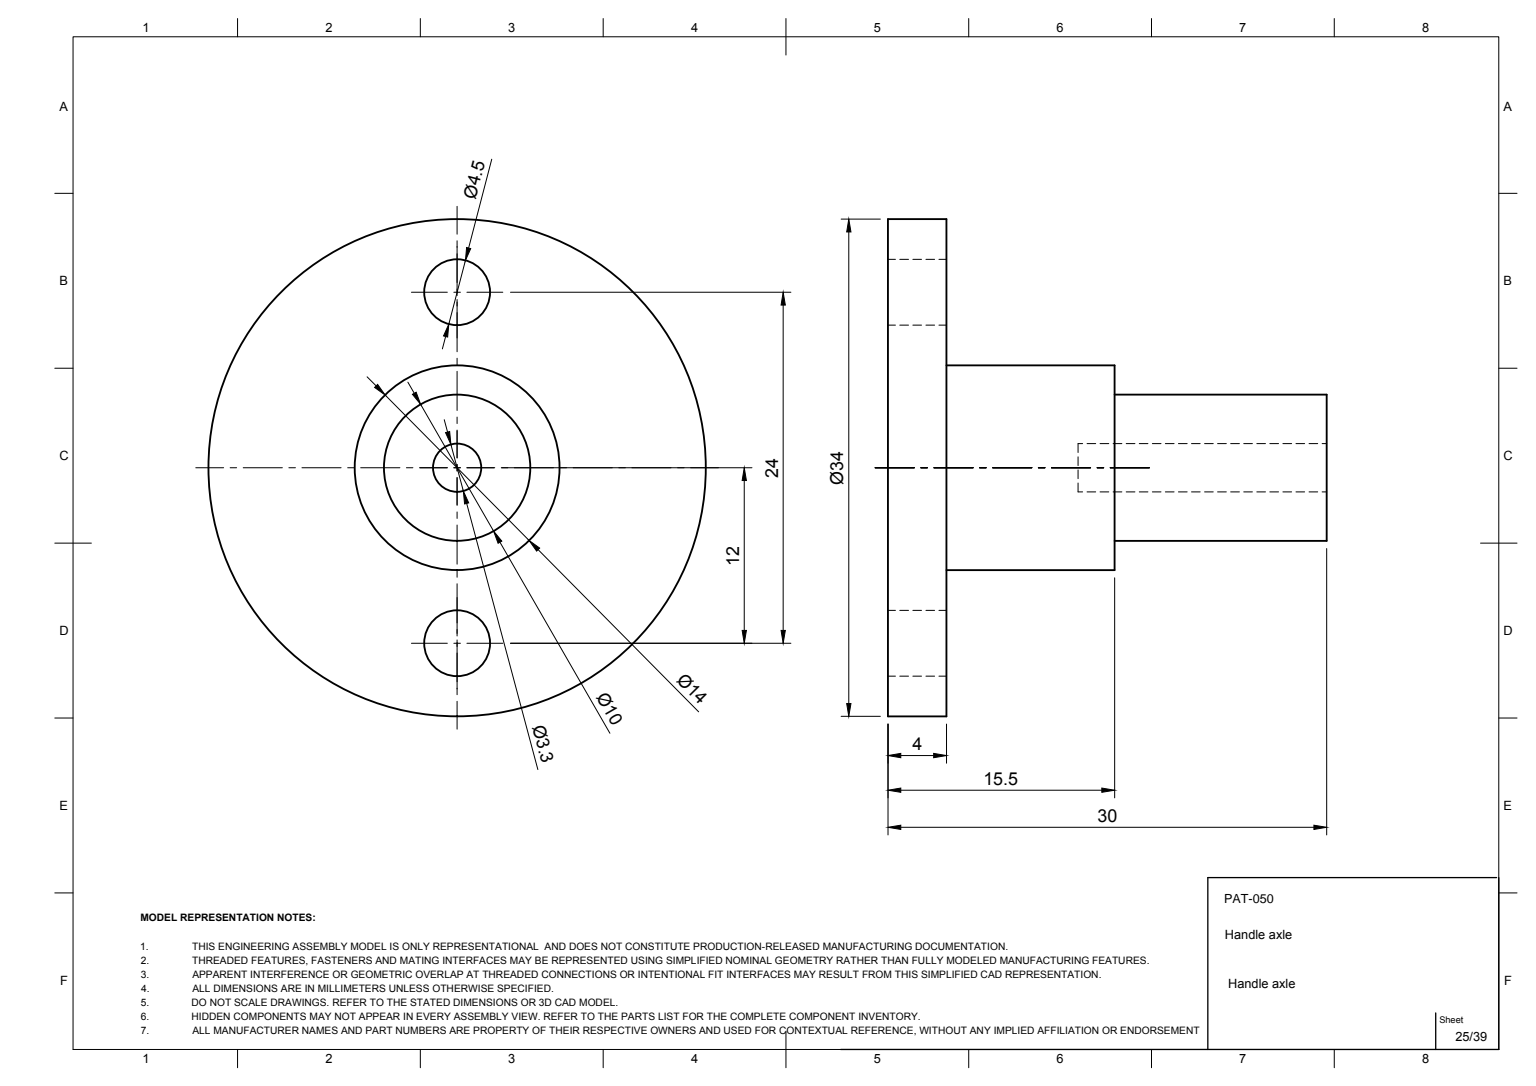
ISO-10303-21;
HEADER;
/* Generated by software containing ST-Developer
 * from STEP Tools, Inc. (www.steptools.com) 
 */

FILE_DESCRIPTION(
/* description */ ('Hand wheel with handle and shaft collar'),
/* implementation_level */ '2;1');

FILE_NAME(
/* name */ 'Handle axle.step',
/* time_stamp */ '2026-10-28T03:23:19-07:00',
/* author */ (''),
/* organization */ (''),
/* preprocessor_version */ 'ST-DEVELOPER v20.2',
/* originating_system */ 'Autodesk Translation Framework v15.17.0.0',
/* authorisation */ '');

FILE_SCHEMA (('AUTOMOTIVE_DESIGN { 1 0 10303 214 3 1 1 }'));
ENDSEC;

DATA;
#10=MECHANICAL_DESIGN_GEOMETRIC_PRESENTATION_REPRESENTATION('',(#420),#10510);
#349=SHAPE_REPRESENTATION_RELATIONSHIP('SRR','None',#10667,#381);
#381=ADVANCED_BREP_SHAPE_REPRESENTATION('',(#466),#10494);
#420=STYLED_ITEM('',(#10908),#466);
#466=MANIFOLD_SOLID_BREP('Body1',#5320);
#570=FACE_BOUND('',#1351,.T.);
#571=FACE_BOUND('',#1352,.T.);
#572=FACE_BOUND('',#1353,.T.);
#573=FACE_BOUND('',#1356,.T.);
#574=FACE_BOUND('',#1360,.T.);
#575=FACE_BOUND('',#1361,.T.);
#576=FACE_BOUND('',#1363,.T.);
#693=PLANE('',#6090);
#694=PLANE('',#6097);
#695=PLANE('',#6102);
#696=PLANE('',#6108);
#697=PLANE('',#6109);
#943=FACE_OUTER_BOUND('',#1346,.T.);
#944=FACE_OUTER_BOUND('',#1347,.T.);
#945=FACE_OUTER_BOUND('',#1348,.T.);
#946=FACE_OUTER_BOUND('',#1349,.T.);
#947=FACE_OUTER_BOUND('',#1350,.T.);
#948=FACE_OUTER_BOUND('',#1354,.T.);
#949=FACE_OUTER_BOUND('',#1355,.T.);
#950=FACE_OUTER_BOUND('',#1357,.T.);
#951=FACE_OUTER_BOUND('',#1358,.T.);
#952=FACE_OUTER_BOUND('',#1359,.T.);
#953=FACE_OUTER_BOUND('',#1362,.T.);
#1346=EDGE_LOOP('',(#4347,#4348,#4349,#4350));
#1347=EDGE_LOOP('',(#4351));
#1348=EDGE_LOOP('',(#4352,#4353,#4354,#4355));
#1349=EDGE_LOOP('',(#4356,#4357,#4358,#4359));
#1350=EDGE_LOOP('',(#4360));
#1351=EDGE_LOOP('',(#4361));
#1352=EDGE_LOOP('',(#4362));
#1353=EDGE_LOOP('',(#4363));
#1354=EDGE_LOOP('',(#4364,#4365,#4366,#4367));
#1355=EDGE_LOOP('',(#4368));
#1356=EDGE_LOOP('',(#4369));
#1357=EDGE_LOOP('',(#4370,#4371,#4372,#4373));
#1358=EDGE_LOOP('',(#4374,#4375,#4376,#4377));
#1359=EDGE_LOOP('',(#4378));
#1360=EDGE_LOOP('',(#4379));
#1361=EDGE_LOOP('',(#4380));
#1362=EDGE_LOOP('',(#4381));
#1363=EDGE_LOOP('',(#4382));
#1704=LINE('',#9449,#2014);
#1705=LINE('',#9456,#2015);
#1706=LINE('',#9462,#2016);
#1707=LINE('',#9472,#2017);
#1708=LINE('',#9479,#2018);
#1709=LINE('',#9482,#2019);
#2014=VECTOR('',#7394,0.165);
#2015=VECTOR('',#7403,0.225);
#2016=VECTOR('',#7410,0.225);
#2017=VECTOR('',#7423,1.7);
#2018=VECTOR('',#7432,0.7);
#2019=VECTOR('',#7435,0.5);
#2315=CIRCLE('',#6088,0.165);
#2316=CIRCLE('',#6089,0.165);
#2317=CIRCLE('',#6092,0.225);
#2318=CIRCLE('',#6093,0.225);
#2319=CIRCLE('',#6095,0.225);
#2320=CIRCLE('',#6096,0.225);
#2321=CIRCLE('',#6098,1.7);
#2322=CIRCLE('',#6099,0.7);
#2323=CIRCLE('',#6101,1.7);
#2324=CIRCLE('',#6103,0.7);
#2325=CIRCLE('',#6104,0.5);
#2326=CIRCLE('',#6107,0.5);
#2715=VERTEX_POINT('',#9446);
#2716=VERTEX_POINT('',#9448);
#2717=VERTEX_POINT('',#9453);
#2718=VERTEX_POINT('',#9455);
#2719=VERTEX_POINT('',#9459);
#2720=VERTEX_POINT('',#9461);
#2721=VERTEX_POINT('',#9465);
#2722=VERTEX_POINT('',#9467);
#2723=VERTEX_POINT('',#9470);
#2724=VERTEX_POINT('',#9474);
#2725=VERTEX_POINT('',#9476);
#2726=VERTEX_POINT('',#9481);
#3291=EDGE_CURVE('',#2715,#2715,#2315,.T.);
#3292=EDGE_CURVE('',#2715,#2716,#1704,.T.);
#3293=EDGE_CURVE('',#2716,#2716,#2316,.T.);
#3294=EDGE_CURVE('',#2717,#2717,#2317,.T.);
#3295=EDGE_CURVE('',#2717,#2718,#1705,.T.);
#3296=EDGE_CURVE('',#2718,#2718,#2318,.T.);
#3297=EDGE_CURVE('',#2719,#2719,#2319,.T.);
#3298=EDGE_CURVE('',#2719,#2720,#1706,.T.);
#3299=EDGE_CURVE('',#2720,#2720,#2320,.T.);
#3300=EDGE_CURVE('',#2721,#2721,#2321,.T.);
#3301=EDGE_CURVE('',#2722,#2722,#2322,.T.);
#3302=EDGE_CURVE('',#2723,#2723,#2323,.T.);
#3303=EDGE_CURVE('',#2723,#2721,#1707,.T.);
#3304=EDGE_CURVE('',#2724,#2724,#2324,.T.);
#3305=EDGE_CURVE('',#2725,#2725,#2325,.T.);
#3306=EDGE_CURVE('',#2722,#2724,#1708,.T.);
#3307=EDGE_CURVE('',#2725,#2726,#1709,.T.);
#3308=EDGE_CURVE('',#2726,#2726,#2326,.T.);
#4347=ORIENTED_EDGE('',*,*,#3291,.F.);
#4348=ORIENTED_EDGE('',*,*,#3292,.T.);
#4349=ORIENTED_EDGE('',*,*,#3293,.T.);
#4350=ORIENTED_EDGE('',*,*,#3292,.F.);
#4351=ORIENTED_EDGE('',*,*,#3293,.F.);
#4352=ORIENTED_EDGE('',*,*,#3294,.F.);
#4353=ORIENTED_EDGE('',*,*,#3295,.T.);
#4354=ORIENTED_EDGE('',*,*,#3296,.F.);
#4355=ORIENTED_EDGE('',*,*,#3295,.F.);
#4356=ORIENTED_EDGE('',*,*,#3297,.F.);
#4357=ORIENTED_EDGE('',*,*,#3298,.T.);
#4358=ORIENTED_EDGE('',*,*,#3299,.F.);
#4359=ORIENTED_EDGE('',*,*,#3298,.F.);
#4360=ORIENTED_EDGE('',*,*,#3300,.F.);
#4361=ORIENTED_EDGE('',*,*,#3294,.T.);
#4362=ORIENTED_EDGE('',*,*,#3297,.T.);
#4363=ORIENTED_EDGE('',*,*,#3301,.F.);
#4364=ORIENTED_EDGE('',*,*,#3302,.F.);
#4365=ORIENTED_EDGE('',*,*,#3303,.T.);
#4366=ORIENTED_EDGE('',*,*,#3300,.T.);
#4367=ORIENTED_EDGE('',*,*,#3303,.F.);
#4368=ORIENTED_EDGE('',*,*,#3304,.F.);
#4369=ORIENTED_EDGE('',*,*,#3305,.F.);
#4370=ORIENTED_EDGE('',*,*,#3301,.T.);
#4371=ORIENTED_EDGE('',*,*,#3306,.T.);
#4372=ORIENTED_EDGE('',*,*,#3304,.T.);
#4373=ORIENTED_EDGE('',*,*,#3306,.F.);
#4374=ORIENTED_EDGE('',*,*,#3305,.T.);
#4375=ORIENTED_EDGE('',*,*,#3307,.T.);
#4376=ORIENTED_EDGE('',*,*,#3308,.T.);
#4377=ORIENTED_EDGE('',*,*,#3307,.F.);
#4378=ORIENTED_EDGE('',*,*,#3302,.T.);
#4379=ORIENTED_EDGE('',*,*,#3296,.T.);
#4380=ORIENTED_EDGE('',*,*,#3299,.T.);
#4381=ORIENTED_EDGE('',*,*,#3308,.F.);
#4382=ORIENTED_EDGE('',*,*,#3291,.T.);
#4941=CYLINDRICAL_SURFACE('',#6087,0.165);
#4942=CYLINDRICAL_SURFACE('',#6091,0.225);
#4943=CYLINDRICAL_SURFACE('',#6094,0.225);
#4944=CYLINDRICAL_SURFACE('',#6100,1.7);
#4945=CYLINDRICAL_SURFACE('',#6105,0.7);
#4946=CYLINDRICAL_SURFACE('',#6106,0.5);
#5155=ADVANCED_FACE('',(#943),#4941,.F.);
#5156=ADVANCED_FACE('',(#944),#693,.F.);
#5157=ADVANCED_FACE('',(#945),#4942,.F.);
#5158=ADVANCED_FACE('',(#946),#4943,.F.);
#5159=ADVANCED_FACE('',(#947,#570,#571,#572),#694,.F.);
#5160=ADVANCED_FACE('',(#948),#4944,.T.);
#5161=ADVANCED_FACE('',(#949,#573),#695,.F.);
#5162=ADVANCED_FACE('',(#950),#4945,.T.);
#5163=ADVANCED_FACE('',(#951),#4946,.T.);
#5164=ADVANCED_FACE('',(#952,#574,#575),#696,.T.);
#5165=ADVANCED_FACE('',(#953,#576),#697,.F.);
#5320=CLOSED_SHELL('',(#5155,#5156,#5157,#5158,#5159,#5160,#5161,#5162,
#5163,#5164,#5165));
#6086=AXIS2_PLACEMENT_3D('',#9444,#7388,#7389);
#6087=AXIS2_PLACEMENT_3D('',#9445,#7390,#7391);
#6088=AXIS2_PLACEMENT_3D('',#9447,#7392,#7393);
#6089=AXIS2_PLACEMENT_3D('',#9450,#7395,#7396);
#6090=AXIS2_PLACEMENT_3D('',#9451,#7397,#7398);
#6091=AXIS2_PLACEMENT_3D('',#9452,#7399,#7400);
#6092=AXIS2_PLACEMENT_3D('',#9454,#7401,#7402);
#6093=AXIS2_PLACEMENT_3D('',#9457,#7404,#7405);
#6094=AXIS2_PLACEMENT_3D('',#9458,#7406,#7407);
#6095=AXIS2_PLACEMENT_3D('',#9460,#7408,#7409);
#6096=AXIS2_PLACEMENT_3D('',#9463,#7411,#7412);
#6097=AXIS2_PLACEMENT_3D('',#9464,#7413,#7414);
#6098=AXIS2_PLACEMENT_3D('',#9466,#7415,#7416);
#6099=AXIS2_PLACEMENT_3D('',#9468,#7417,#7418);
#6100=AXIS2_PLACEMENT_3D('',#9469,#7419,#7420);
#6101=AXIS2_PLACEMENT_3D('',#9471,#7421,#7422);
#6102=AXIS2_PLACEMENT_3D('',#9473,#7424,#7425);
#6103=AXIS2_PLACEMENT_3D('',#9475,#7426,#7427);
#6104=AXIS2_PLACEMENT_3D('',#9477,#7428,#7429);
#6105=AXIS2_PLACEMENT_3D('',#9478,#7430,#7431);
#6106=AXIS2_PLACEMENT_3D('',#9480,#7433,#7434);
#6107=AXIS2_PLACEMENT_3D('',#9483,#7436,#7437);
#6108=AXIS2_PLACEMENT_3D('',#9484,#7438,#7439);
#6109=AXIS2_PLACEMENT_3D('',#9485,#7440,#7441);
#7388=DIRECTION('axis',(0.,0.,1.));
#7389=DIRECTION('refdir',(1.,0.,0.));
#7390=DIRECTION('center_axis',(0.,1.,0.));
#7391=DIRECTION('ref_axis',(1.,0.,0.));
#7392=DIRECTION('center_axis',(0.,1.,0.));
#7393=DIRECTION('ref_axis',(1.,0.,0.));
#7394=DIRECTION('',(0.,1.,0.));
#7395=DIRECTION('center_axis',(0.,1.,0.));
#7396=DIRECTION('ref_axis',(1.,0.,0.));
#7397=DIRECTION('center_axis',(0.,1.,0.));
#7398=DIRECTION('ref_axis',(1.,0.,0.));
#7399=DIRECTION('center_axis',(0.,1.,0.));
#7400=DIRECTION('ref_axis',(1.,0.,0.));
#7401=DIRECTION('center_axis',(0.,1.,0.));
#7402=DIRECTION('ref_axis',(1.,0.,0.));
#7403=DIRECTION('',(0.,1.,0.));
#7404=DIRECTION('center_axis',(0.,-1.,0.));
#7405=DIRECTION('ref_axis',(1.,0.,0.));
#7406=DIRECTION('center_axis',(0.,1.,0.));
#7407=DIRECTION('ref_axis',(1.,0.,0.));
#7408=DIRECTION('center_axis',(0.,1.,0.));
#7409=DIRECTION('ref_axis',(1.,0.,0.));
#7410=DIRECTION('',(0.,1.,0.));
#7411=DIRECTION('center_axis',(0.,-1.,0.));
#7412=DIRECTION('ref_axis',(1.,0.,0.));
#7413=DIRECTION('center_axis',(0.,1.,0.));
#7414=DIRECTION('ref_axis',(1.,0.,0.));
#7415=DIRECTION('center_axis',(0.,1.,0.));
#7416=DIRECTION('ref_axis',(1.,0.,0.));
#7417=DIRECTION('center_axis',(0.,-1.,0.));
#7418=DIRECTION('ref_axis',(1.,0.,0.));
#7419=DIRECTION('center_axis',(0.,1.,0.));
#7420=DIRECTION('ref_axis',(1.,0.,0.));
#7421=DIRECTION('center_axis',(0.,1.,0.));
#7422=DIRECTION('ref_axis',(1.,0.,0.));
#7423=DIRECTION('',(0.,-1.,0.));
#7424=DIRECTION('center_axis',(0.,1.,0.));
#7425=DIRECTION('ref_axis',(1.,0.,0.));
#7426=DIRECTION('center_axis',(0.,1.,0.));
#7427=DIRECTION('ref_axis',(1.,0.,0.));
#7428=DIRECTION('center_axis',(0.,-1.,0.));
#7429=DIRECTION('ref_axis',(1.,0.,0.));
#7430=DIRECTION('center_axis',(0.,1.,0.));
#7431=DIRECTION('ref_axis',(1.,0.,0.));
#7432=DIRECTION('',(0.,-1.,0.));
#7433=DIRECTION('center_axis',(0.,1.,0.));
#7434=DIRECTION('ref_axis',(1.,0.,0.));
#7435=DIRECTION('',(0.,-1.,0.));
#7436=DIRECTION('center_axis',(0.,1.,0.));
#7437=DIRECTION('ref_axis',(1.,0.,0.));
#7438=DIRECTION('center_axis',(0.,1.,0.));
#7439=DIRECTION('ref_axis',(1.,0.,0.));
#7440=DIRECTION('center_axis',(0.,1.,0.));
#7441=DIRECTION('ref_axis',(1.,0.,0.));
#9444=CARTESIAN_POINT('',(0.,0.,0.));
#9445=CARTESIAN_POINT('Origin',(6.5,-6.1,10.));
#9446=CARTESIAN_POINT('',(6.335,-6.,10.));
#9447=CARTESIAN_POINT('Origin',(6.5,-6.,10.));
#9448=CARTESIAN_POINT('',(6.335,-4.3,10.));
#9449=CARTESIAN_POINT('',(6.335,-6.1,10.));
#9450=CARTESIAN_POINT('Origin',(6.5,-4.3,10.));
#9451=CARTESIAN_POINT('Origin',(6.5,-4.3,10.));
#9452=CARTESIAN_POINT('Origin',(5.3,-3.5,10.));
#9453=CARTESIAN_POINT('',(5.075,-3.4,10.));
#9454=CARTESIAN_POINT('Origin',(5.3,-3.4,10.));
#9455=CARTESIAN_POINT('',(5.075,-3.,10.));
#9456=CARTESIAN_POINT('',(5.075,-3.5,10.));
#9457=CARTESIAN_POINT('Origin',(5.3,-3.,10.));
#9458=CARTESIAN_POINT('Origin',(7.7,-3.5,10.));
#9459=CARTESIAN_POINT('',(7.475,-3.4,10.));
#9460=CARTESIAN_POINT('Origin',(7.7,-3.4,10.));
#9461=CARTESIAN_POINT('',(7.475,-3.,10.));
#9462=CARTESIAN_POINT('',(7.475,-3.5,10.));
#9463=CARTESIAN_POINT('Origin',(7.7,-3.,10.));
#9464=CARTESIAN_POINT('Origin',(6.5,-3.4,10.));
#9465=CARTESIAN_POINT('',(4.8,-3.4,10.));
#9466=CARTESIAN_POINT('Origin',(6.5,-3.4,10.));
#9467=CARTESIAN_POINT('',(5.8,-3.4,10.));
#9468=CARTESIAN_POINT('Origin',(6.5,-3.4,10.));
#9469=CARTESIAN_POINT('Origin',(6.5,-3.4,10.));
#9470=CARTESIAN_POINT('',(4.8,-3.,10.));
#9471=CARTESIAN_POINT('Origin',(6.5,-3.,10.));
#9472=CARTESIAN_POINT('',(4.8,-3.4,10.));
#9473=CARTESIAN_POINT('Origin',(6.5,-4.55,10.));
#9474=CARTESIAN_POINT('',(5.8,-4.55,10.));
#9475=CARTESIAN_POINT('Origin',(6.5,-4.55,10.));
#9476=CARTESIAN_POINT('',(6.,-4.55,10.));
#9477=CARTESIAN_POINT('Origin',(6.5,-4.55,10.));
#9478=CARTESIAN_POINT('Origin',(6.5,-4.55,10.));
#9479=CARTESIAN_POINT('',(5.8,-4.55,10.));
#9480=CARTESIAN_POINT('Origin',(6.5,-6.,10.));
#9481=CARTESIAN_POINT('',(6.,-6.,10.));
#9482=CARTESIAN_POINT('',(6.,-6.,10.));
#9483=CARTESIAN_POINT('Origin',(6.5,-6.,10.));
#9484=CARTESIAN_POINT('Origin',(6.5,-3.,10.));
#9485=CARTESIAN_POINT('Origin',(6.5,-6.,10.));
#10455=UNCERTAINTY_MEASURE_WITH_UNIT(LENGTH_MEASURE(0.001),#10511,
'DISTANCE_ACCURACY_VALUE',
'Maximum model space distance between geometric entities at asserted c
onnectivities');
#10471=UNCERTAINTY_MEASURE_WITH_UNIT(LENGTH_MEASURE(0.001),#10511,
'DISTANCE_ACCURACY_VALUE',
'Maximum model space distance between geometric entities at asserted c
onnectivities');
#10494=(
GEOMETRIC_REPRESENTATION_CONTEXT(3)
GLOBAL_UNCERTAINTY_ASSIGNED_CONTEXT((#10455))
GLOBAL_UNIT_ASSIGNED_CONTEXT((#10511,#10513,#10514))
REPRESENTATION_CONTEXT('','3D')
);
#10510=(
GEOMETRIC_REPRESENTATION_CONTEXT(3)
GLOBAL_UNCERTAINTY_ASSIGNED_CONTEXT((#10471))
GLOBAL_UNIT_ASSIGNED_CONTEXT((#10511,#10513,#10514))
REPRESENTATION_CONTEXT('','3D')
);
#10511=(
LENGTH_UNIT()
NAMED_UNIT(*)
SI_UNIT(.CENTI.,.METRE.)
);
#10513=(
NAMED_UNIT(*)
PLANE_ANGLE_UNIT()
SI_UNIT($,.RADIAN.)
);
#10514=(
NAMED_UNIT(*)
SI_UNIT($,.STERADIAN.)
SOLID_ANGLE_UNIT()
);
#10537=SHAPE_DEFINITION_REPRESENTATION(#10580,#10667);
#10580=PRODUCT_DEFINITION_SHAPE('',$,#10706);
#10667=SHAPE_REPRESENTATION('',(#6086),#10494);
#10683=PRODUCT_DEFINITION_CONTEXT('part definition',#10799,'design');
#10706=PRODUCT_DEFINITION('Handle axle','Handle axle',#10744,#10683);
#10744=PRODUCT_DEFINITION_FORMATION('',$,#10823);
#10799=APPLICATION_CONTEXT(
'Core Data for Automotive Mechanical Design Process');
#10800=PRODUCT_CONTEXT('part definition',#10799,'mechanical');
#10823=PRODUCT('Handle axle','Handle axle','Handle axle',(#10800));
#10902=COLOUR_RGB('Grey',0.48,0.52,0.57);
#10903=FILL_AREA_STYLE_COLOUR('',#10902);
#10904=FILL_AREA_STYLE('',(#10903));
#10905=SURFACE_STYLE_FILL_AREA(#10904);
#10906=SURFACE_SIDE_STYLE('',(#10905));
#10907=SURFACE_STYLE_USAGE(.BOTH.,#10906);
#10908=PRESENTATION_STYLE_ASSIGNMENT((#10907));
ENDSEC;
END-ISO-10303-21;
